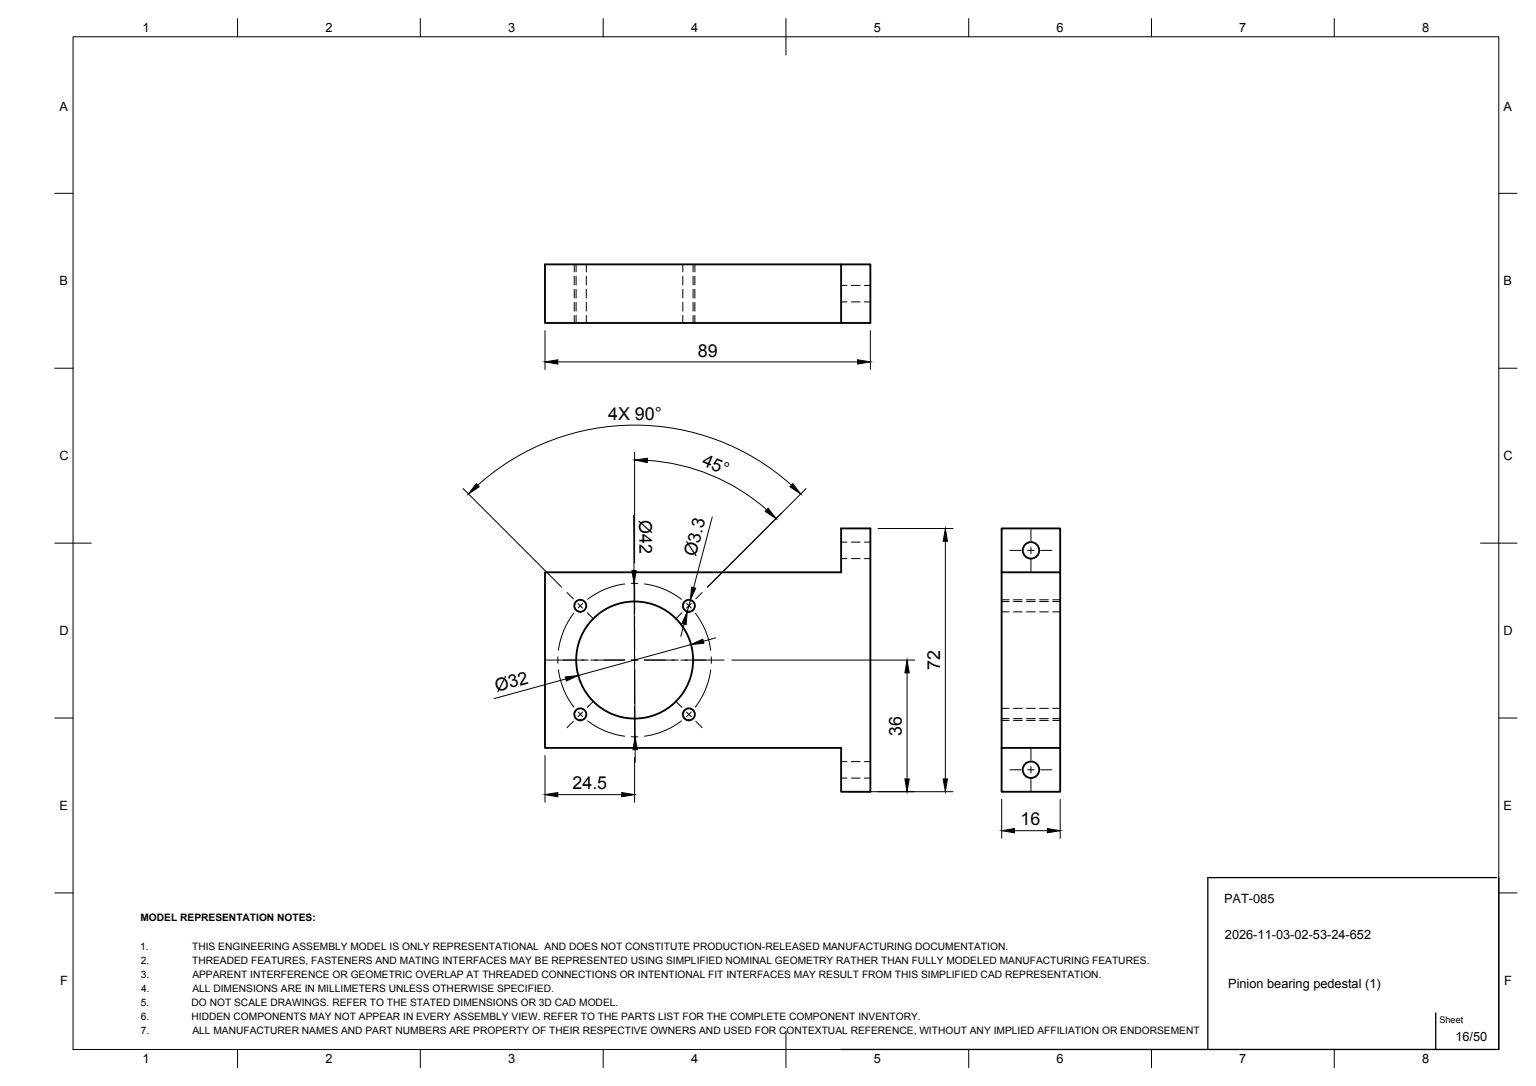
ISO-10303-21;
HEADER;
/* Generated by software containing ST-Developer
 * from STEP Tools, Inc. (www.steptools.com) 
 */

FILE_DESCRIPTION(
/* description */ ('Rack and pinion manual slide'),
/* implementation_level */ '2;1');

FILE_NAME(
/* name */ 'Pinion bearing pedestal (1).step',
/* time_stamp */ '2026-10-28T03:22:49-07:00',
/* author */ (''),
/* organization */ (''),
/* preprocessor_version */ 'ST-DEVELOPER v20.2',
/* originating_system */ 'Autodesk Translation Framework v15.17.0.0',
/* authorisation */ '');

FILE_SCHEMA (('AUTOMOTIVE_DESIGN { 1 0 10303 214 3 1 1 }'));
ENDSEC;

DATA;
#10=MECHANICAL_DESIGN_GEOMETRIC_PRESENTATION_REPRESENTATION('',(#743),#34851);
#651=SHAPE_REPRESENTATION_RELATIONSHIP('SRR','None',#35086,#697);
#697=ADVANCED_BREP_SHAPE_REPRESENTATION('',(#796),#34811);
#743=STYLED_ITEM('',(#35411),#796);
#796=MANIFOLD_SOLID_BREP('Body1',#13763);
#921=FACE_BOUND('',#2487,.T.);
#922=FACE_BOUND('',#2489,.T.);
#923=FACE_BOUND('',#2493,.T.);
#924=FACE_BOUND('',#2494,.T.);
#925=FACE_BOUND('',#2495,.T.);
#926=FACE_BOUND('',#2496,.T.);
#927=FACE_BOUND('',#2497,.T.);
#928=FACE_BOUND('',#2500,.T.);
#929=FACE_BOUND('',#2501,.T.);
#930=FACE_BOUND('',#2502,.T.);
#931=FACE_BOUND('',#2503,.T.);
#932=FACE_BOUND('',#2504,.T.);
#933=FACE_BOUND('',#2508,.T.);
#934=FACE_BOUND('',#2509,.T.);
#1112=PLANE('',#14567);
#1113=PLANE('',#14568);
#1114=PLANE('',#14569);
#1115=PLANE('',#14570);
#1116=PLANE('',#14571);
#1117=PLANE('',#14572);
#1118=PLANE('',#14573);
#1119=PLANE('',#14574);
#1120=PLANE('',#14575);
#1121=PLANE('',#14576);
#1652=FACE_OUTER_BOUND('',#2479,.T.);
#1653=FACE_OUTER_BOUND('',#2480,.T.);
#1654=FACE_OUTER_BOUND('',#2481,.T.);
#1655=FACE_OUTER_BOUND('',#2482,.T.);
#1656=FACE_OUTER_BOUND('',#2483,.T.);
#1657=FACE_OUTER_BOUND('',#2484,.T.);
#1658=FACE_OUTER_BOUND('',#2485,.T.);
#1659=FACE_OUTER_BOUND('',#2486,.T.);
#1660=FACE_OUTER_BOUND('',#2488,.T.);
#1661=FACE_OUTER_BOUND('',#2490,.T.);
#1662=FACE_OUTER_BOUND('',#2491,.T.);
#1663=FACE_OUTER_BOUND('',#2492,.T.);
#1664=FACE_OUTER_BOUND('',#2498,.T.);
#1665=FACE_OUTER_BOUND('',#2499,.T.);
#1666=FACE_OUTER_BOUND('',#2505,.T.);
#1667=FACE_OUTER_BOUND('',#2506,.T.);
#1668=FACE_OUTER_BOUND('',#2507,.T.);
#2479=EDGE_LOOP('',(#9768,#9769,#9770,#9771));
#2480=EDGE_LOOP('',(#9772,#9773,#9774,#9775));
#2481=EDGE_LOOP('',(#9776,#9777,#9778,#9779));
#2482=EDGE_LOOP('',(#9780,#9781,#9782,#9783));
#2483=EDGE_LOOP('',(#9784,#9785,#9786,#9787));
#2484=EDGE_LOOP('',(#9788,#9789,#9790,#9791));
#2485=EDGE_LOOP('',(#9792,#9793,#9794,#9795));
#2486=EDGE_LOOP('',(#9796,#9797,#9798,#9799));
#2487=EDGE_LOOP('',(#9800));
#2488=EDGE_LOOP('',(#9801,#9802,#9803,#9804));
#2489=EDGE_LOOP('',(#9805));
#2490=EDGE_LOOP('',(#9806,#9807,#9808,#9809));
#2491=EDGE_LOOP('',(#9810,#9811,#9812,#9813));
#2492=EDGE_LOOP('',(#9814,#9815,#9816,#9817,#9818,#9819,#9820,#9821));
#2493=EDGE_LOOP('',(#9822));
#2494=EDGE_LOOP('',(#9823));
#2495=EDGE_LOOP('',(#9824));
#2496=EDGE_LOOP('',(#9825));
#2497=EDGE_LOOP('',(#9826));
#2498=EDGE_LOOP('',(#9827,#9828,#9829,#9830));
#2499=EDGE_LOOP('',(#9831,#9832,#9833,#9834,#9835,#9836,#9837,#9838));
#2500=EDGE_LOOP('',(#9839));
#2501=EDGE_LOOP('',(#9840));
#2502=EDGE_LOOP('',(#9841));
#2503=EDGE_LOOP('',(#9842));
#2504=EDGE_LOOP('',(#9843));
#2505=EDGE_LOOP('',(#9844,#9845,#9846,#9847));
#2506=EDGE_LOOP('',(#9848,#9849,#9850,#9851));
#2507=EDGE_LOOP('',(#9852,#9853,#9854,#9855));
#2508=EDGE_LOOP('',(#9856));
#2509=EDGE_LOOP('',(#9857));
#3393=LINE('',#20037,#4684);
#3394=LINE('',#20043,#4685);
#3395=LINE('',#20049,#4686);
#3396=LINE('',#20055,#4687);
#3397=LINE('',#20061,#4688);
#3398=LINE('',#20067,#4689);
#3399=LINE('',#20073,#4690);
#3400=LINE('',#20078,#4691);
#3401=LINE('',#20080,#4692);
#3402=LINE('',#20082,#4693);
#3403=LINE('',#20083,#4694);
#3404=LINE('',#20087,#4695);
#3405=LINE('',#20089,#4696);
#3406=LINE('',#20091,#4697);
#3407=LINE('',#20092,#4698);
#3408=LINE('',#20095,#4699);
#3409=LINE('',#20097,#4700);
#3410=LINE('',#20098,#4701);
#3411=LINE('',#20101,#4702);
#3412=LINE('',#20103,#4703);
#3413=LINE('',#20104,#4704);
#3414=LINE('',#20107,#4705);
#3415=LINE('',#20109,#4706);
#3416=LINE('',#20110,#4707);
#3417=LINE('',#20111,#4708);
#3418=LINE('',#20114,#4709);
#3419=LINE('',#20115,#4710);
#3420=LINE('',#20118,#4711);
#3421=LINE('',#20119,#4712);
#3422=LINE('',#20120,#4713);
#3423=LINE('',#20122,#4714);
#4684=VECTOR('',#16231,0.225);
#4685=VECTOR('',#16238,0.225);
#4686=VECTOR('',#16245,0.164999999999999);
#4687=VECTOR('',#16252,0.164999999999999);
#4688=VECTOR('',#16259,0.164999999999999);
#4689=VECTOR('',#16266,0.164999999999999);
#4690=VECTOR('',#16273,1.6);
#4691=VECTOR('',#16278,1.);
#4692=VECTOR('',#16279,1.);
#4693=VECTOR('',#16280,1.);
#4694=VECTOR('',#16281,1.);
#4695=VECTOR('',#16284,1.);
#4696=VECTOR('',#16285,1.);
#4697=VECTOR('',#16286,1.);
#4698=VECTOR('',#16287,1.);
#4699=VECTOR('',#16290,1.);
#4700=VECTOR('',#16291,1.);
#4701=VECTOR('',#16292,1.);
#4702=VECTOR('',#16295,1.);
#4703=VECTOR('',#16296,1.);
#4704=VECTOR('',#16297,1.);
#4705=VECTOR('',#16300,1.);
#4706=VECTOR('',#16301,1.);
#4707=VECTOR('',#16302,1.);
#4708=VECTOR('',#16303,1.);
#4709=VECTOR('',#16306,1.);
#4710=VECTOR('',#16307,1.);
#4711=VECTOR('',#16310,1.);
#4712=VECTOR('',#16311,1.);
#4713=VECTOR('',#16312,1.);
#4714=VECTOR('',#16315,1.);
#5904=CIRCLE('',#14547,0.225);
#5905=CIRCLE('',#14548,0.225);
#5906=CIRCLE('',#14550,0.225);
#5907=CIRCLE('',#14551,0.225);
#5908=CIRCLE('',#14553,0.164999999999999);
#5909=CIRCLE('',#14554,0.164999999999999);
#5910=CIRCLE('',#14556,0.164999999999999);
#5911=CIRCLE('',#14557,0.164999999999999);
#5912=CIRCLE('',#14559,0.164999999999999);
#5913=CIRCLE('',#14560,0.164999999999999);
#5914=CIRCLE('',#14562,0.164999999999999);
#5915=CIRCLE('',#14563,0.164999999999999);
#5916=CIRCLE('',#14565,1.6);
#5917=CIRCLE('',#14566,1.6);
#6402=VERTEX_POINT('',#20034);
#6403=VERTEX_POINT('',#20036);
#6404=VERTEX_POINT('',#20040);
#6405=VERTEX_POINT('',#20042);
#6406=VERTEX_POINT('',#20046);
#6407=VERTEX_POINT('',#20048);
#6408=VERTEX_POINT('',#20052);
#6409=VERTEX_POINT('',#20054);
#6410=VERTEX_POINT('',#20058);
#6411=VERTEX_POINT('',#20060);
#6412=VERTEX_POINT('',#20064);
#6413=VERTEX_POINT('',#20066);
#6414=VERTEX_POINT('',#20070);
#6415=VERTEX_POINT('',#20072);
#6416=VERTEX_POINT('',#20076);
#6417=VERTEX_POINT('',#20077);
#6418=VERTEX_POINT('',#20079);
#6419=VERTEX_POINT('',#20081);
#6420=VERTEX_POINT('',#20085);
#6421=VERTEX_POINT('',#20086);
#6422=VERTEX_POINT('',#20088);
#6423=VERTEX_POINT('',#20090);
#6424=VERTEX_POINT('',#20094);
#6425=VERTEX_POINT('',#20096);
#6426=VERTEX_POINT('',#20100);
#6427=VERTEX_POINT('',#20102);
#6428=VERTEX_POINT('',#20106);
#6429=VERTEX_POINT('',#20108);
#6430=VERTEX_POINT('',#20113);
#6431=VERTEX_POINT('',#20117);
#7696=EDGE_CURVE('',#6402,#6402,#5904,.T.);
#7697=EDGE_CURVE('',#6402,#6403,#3393,.T.);
#7698=EDGE_CURVE('',#6403,#6403,#5905,.T.);
#7699=EDGE_CURVE('',#6404,#6404,#5906,.T.);
#7700=EDGE_CURVE('',#6404,#6405,#3394,.T.);
#7701=EDGE_CURVE('',#6405,#6405,#5907,.T.);
#7702=EDGE_CURVE('',#6406,#6406,#5908,.T.);
#7703=EDGE_CURVE('',#6406,#6407,#3395,.T.);
#7704=EDGE_CURVE('',#6407,#6407,#5909,.T.);
#7705=EDGE_CURVE('',#6408,#6408,#5910,.T.);
#7706=EDGE_CURVE('',#6408,#6409,#3396,.T.);
#7707=EDGE_CURVE('',#6409,#6409,#5911,.T.);
#7708=EDGE_CURVE('',#6410,#6410,#5912,.T.);
#7709=EDGE_CURVE('',#6410,#6411,#3397,.T.);
#7710=EDGE_CURVE('',#6411,#6411,#5913,.T.);
#7711=EDGE_CURVE('',#6412,#6412,#5914,.T.);
#7712=EDGE_CURVE('',#6412,#6413,#3398,.T.);
#7713=EDGE_CURVE('',#6413,#6413,#5915,.T.);
#7714=EDGE_CURVE('',#6414,#6414,#5916,.T.);
#7715=EDGE_CURVE('',#6414,#6415,#3399,.T.);
#7716=EDGE_CURVE('',#6415,#6415,#5917,.T.);
#7717=EDGE_CURVE('',#6416,#6417,#3400,.T.);
#7718=EDGE_CURVE('',#6418,#6416,#3401,.T.);
#7719=EDGE_CURVE('',#6418,#6419,#3402,.T.);
#7720=EDGE_CURVE('',#6417,#6419,#3403,.T.);
#7721=EDGE_CURVE('',#6420,#6421,#3404,.T.);
#7722=EDGE_CURVE('',#6422,#6420,#3405,.T.);
#7723=EDGE_CURVE('',#6423,#6422,#3406,.T.);
#7724=EDGE_CURVE('',#6421,#6423,#3407,.T.);
#7725=EDGE_CURVE('',#6423,#6424,#3408,.T.);
#7726=EDGE_CURVE('',#6425,#6422,#3409,.T.);
#7727=EDGE_CURVE('',#6424,#6425,#3410,.T.);
#7728=EDGE_CURVE('',#6426,#6418,#3411,.T.);
#7729=EDGE_CURVE('',#6426,#6427,#3412,.T.);
#7730=EDGE_CURVE('',#6419,#6427,#3413,.T.);
#7731=EDGE_CURVE('',#6416,#6428,#3414,.T.);
#7732=EDGE_CURVE('',#6429,#6428,#3415,.T.);
#7733=EDGE_CURVE('',#6421,#6429,#3416,.T.);
#7734=EDGE_CURVE('',#6424,#6426,#3417,.T.);
#7735=EDGE_CURVE('',#6417,#6430,#3418,.T.);
#7736=EDGE_CURVE('',#6428,#6430,#3419,.T.);
#7737=EDGE_CURVE('',#6420,#6431,#3420,.T.);
#7738=EDGE_CURVE('',#6430,#6431,#3421,.T.);
#7739=EDGE_CURVE('',#6427,#6425,#3422,.T.);
#7740=EDGE_CURVE('',#6431,#6429,#3423,.T.);
#9768=ORIENTED_EDGE('',*,*,#7696,.F.);
#9769=ORIENTED_EDGE('',*,*,#7697,.T.);
#9770=ORIENTED_EDGE('',*,*,#7698,.F.);
#9771=ORIENTED_EDGE('',*,*,#7697,.F.);
#9772=ORIENTED_EDGE('',*,*,#7699,.F.);
#9773=ORIENTED_EDGE('',*,*,#7700,.T.);
#9774=ORIENTED_EDGE('',*,*,#7701,.F.);
#9775=ORIENTED_EDGE('',*,*,#7700,.F.);
#9776=ORIENTED_EDGE('',*,*,#7702,.F.);
#9777=ORIENTED_EDGE('',*,*,#7703,.T.);
#9778=ORIENTED_EDGE('',*,*,#7704,.F.);
#9779=ORIENTED_EDGE('',*,*,#7703,.F.);
#9780=ORIENTED_EDGE('',*,*,#7705,.F.);
#9781=ORIENTED_EDGE('',*,*,#7706,.T.);
#9782=ORIENTED_EDGE('',*,*,#7707,.F.);
#9783=ORIENTED_EDGE('',*,*,#7706,.F.);
#9784=ORIENTED_EDGE('',*,*,#7708,.F.);
#9785=ORIENTED_EDGE('',*,*,#7709,.T.);
#9786=ORIENTED_EDGE('',*,*,#7710,.F.);
#9787=ORIENTED_EDGE('',*,*,#7709,.F.);
#9788=ORIENTED_EDGE('',*,*,#7711,.F.);
#9789=ORIENTED_EDGE('',*,*,#7712,.T.);
#9790=ORIENTED_EDGE('',*,*,#7713,.F.);
#9791=ORIENTED_EDGE('',*,*,#7712,.F.);
#9792=ORIENTED_EDGE('',*,*,#7714,.F.);
#9793=ORIENTED_EDGE('',*,*,#7715,.T.);
#9794=ORIENTED_EDGE('',*,*,#7716,.F.);
#9795=ORIENTED_EDGE('',*,*,#7715,.F.);
#9796=ORIENTED_EDGE('',*,*,#7717,.F.);
#9797=ORIENTED_EDGE('',*,*,#7718,.F.);
#9798=ORIENTED_EDGE('',*,*,#7719,.T.);
#9799=ORIENTED_EDGE('',*,*,#7720,.F.);
#9800=ORIENTED_EDGE('',*,*,#7701,.T.);
#9801=ORIENTED_EDGE('',*,*,#7721,.F.);
#9802=ORIENTED_EDGE('',*,*,#7722,.F.);
#9803=ORIENTED_EDGE('',*,*,#7723,.F.);
#9804=ORIENTED_EDGE('',*,*,#7724,.F.);
#9805=ORIENTED_EDGE('',*,*,#7698,.T.);
#9806=ORIENTED_EDGE('',*,*,#7725,.F.);
#9807=ORIENTED_EDGE('',*,*,#7723,.T.);
#9808=ORIENTED_EDGE('',*,*,#7726,.F.);
#9809=ORIENTED_EDGE('',*,*,#7727,.F.);
#9810=ORIENTED_EDGE('',*,*,#7728,.F.);
#9811=ORIENTED_EDGE('',*,*,#7729,.T.);
#9812=ORIENTED_EDGE('',*,*,#7730,.F.);
#9813=ORIENTED_EDGE('',*,*,#7719,.F.);
#9814=ORIENTED_EDGE('',*,*,#7731,.T.);
#9815=ORIENTED_EDGE('',*,*,#7732,.F.);
#9816=ORIENTED_EDGE('',*,*,#7733,.F.);
#9817=ORIENTED_EDGE('',*,*,#7724,.T.);
#9818=ORIENTED_EDGE('',*,*,#7725,.T.);
#9819=ORIENTED_EDGE('',*,*,#7734,.T.);
#9820=ORIENTED_EDGE('',*,*,#7728,.T.);
#9821=ORIENTED_EDGE('',*,*,#7718,.T.);
#9822=ORIENTED_EDGE('',*,*,#7714,.T.);
#9823=ORIENTED_EDGE('',*,*,#7711,.T.);
#9824=ORIENTED_EDGE('',*,*,#7708,.T.);
#9825=ORIENTED_EDGE('',*,*,#7705,.T.);
#9826=ORIENTED_EDGE('',*,*,#7702,.T.);
#9827=ORIENTED_EDGE('',*,*,#7717,.T.);
#9828=ORIENTED_EDGE('',*,*,#7735,.T.);
#9829=ORIENTED_EDGE('',*,*,#7736,.F.);
#9830=ORIENTED_EDGE('',*,*,#7731,.F.);
#9831=ORIENTED_EDGE('',*,*,#7737,.T.);
#9832=ORIENTED_EDGE('',*,*,#7738,.F.);
#9833=ORIENTED_EDGE('',*,*,#7735,.F.);
#9834=ORIENTED_EDGE('',*,*,#7720,.T.);
#9835=ORIENTED_EDGE('',*,*,#7730,.T.);
#9836=ORIENTED_EDGE('',*,*,#7739,.T.);
#9837=ORIENTED_EDGE('',*,*,#7726,.T.);
#9838=ORIENTED_EDGE('',*,*,#7722,.T.);
#9839=ORIENTED_EDGE('',*,*,#7716,.T.);
#9840=ORIENTED_EDGE('',*,*,#7713,.T.);
#9841=ORIENTED_EDGE('',*,*,#7710,.T.);
#9842=ORIENTED_EDGE('',*,*,#7707,.T.);
#9843=ORIENTED_EDGE('',*,*,#7704,.T.);
#9844=ORIENTED_EDGE('',*,*,#7721,.T.);
#9845=ORIENTED_EDGE('',*,*,#7733,.T.);
#9846=ORIENTED_EDGE('',*,*,#7740,.F.);
#9847=ORIENTED_EDGE('',*,*,#7737,.F.);
#9848=ORIENTED_EDGE('',*,*,#7740,.T.);
#9849=ORIENTED_EDGE('',*,*,#7732,.T.);
#9850=ORIENTED_EDGE('',*,*,#7736,.T.);
#9851=ORIENTED_EDGE('',*,*,#7738,.T.);
#9852=ORIENTED_EDGE('',*,*,#7739,.F.);
#9853=ORIENTED_EDGE('',*,*,#7729,.F.);
#9854=ORIENTED_EDGE('',*,*,#7734,.F.);
#9855=ORIENTED_EDGE('',*,*,#7727,.T.);
#9856=ORIENTED_EDGE('',*,*,#7696,.T.);
#9857=ORIENTED_EDGE('',*,*,#7699,.T.);
#12893=CYLINDRICAL_SURFACE('',#14546,0.225);
#12894=CYLINDRICAL_SURFACE('',#14549,0.225);
#12895=CYLINDRICAL_SURFACE('',#14552,0.164999999999999);
#12896=CYLINDRICAL_SURFACE('',#14555,0.164999999999999);
#12897=CYLINDRICAL_SURFACE('',#14558,0.164999999999999);
#12898=CYLINDRICAL_SURFACE('',#14561,0.164999999999999);
#12899=CYLINDRICAL_SURFACE('',#14564,1.6);
#13130=ADVANCED_FACE('',(#1652),#12893,.F.);
#13131=ADVANCED_FACE('',(#1653),#12894,.F.);
#13132=ADVANCED_FACE('',(#1654),#12895,.F.);
#13133=ADVANCED_FACE('',(#1655),#12896,.F.);
#13134=ADVANCED_FACE('',(#1656),#12897,.F.);
#13135=ADVANCED_FACE('',(#1657),#12898,.F.);
#13136=ADVANCED_FACE('',(#1658),#12899,.F.);
#13137=ADVANCED_FACE('',(#1659,#921),#1112,.T.);
#13138=ADVANCED_FACE('',(#1660,#922),#1113,.T.);
#13139=ADVANCED_FACE('',(#1661),#1114,.T.);
#13140=ADVANCED_FACE('',(#1662),#1115,.T.);
#13141=ADVANCED_FACE('',(#1663,#923,#924,#925,#926,#927),#1116,.T.);
#13142=ADVANCED_FACE('',(#1664),#1117,.T.);
#13143=ADVANCED_FACE('',(#1665,#928,#929,#930,#931,#932),#1118,.T.);
#13144=ADVANCED_FACE('',(#1666),#1119,.T.);
#13145=ADVANCED_FACE('',(#1667),#1120,.T.);
#13146=ADVANCED_FACE('',(#1668,#933,#934),#1121,.F.);
#13763=CLOSED_SHELL('',(#13130,#13131,#13132,#13133,#13134,#13135,#13136,
#13137,#13138,#13139,#13140,#13141,#13142,#13143,#13144,#13145,#13146));
#14545=AXIS2_PLACEMENT_3D('',#20032,#16225,#16226);
#14546=AXIS2_PLACEMENT_3D('',#20033,#16227,#16228);
#14547=AXIS2_PLACEMENT_3D('',#20035,#16229,#16230);
#14548=AXIS2_PLACEMENT_3D('',#20038,#16232,#16233);
#14549=AXIS2_PLACEMENT_3D('',#20039,#16234,#16235);
#14550=AXIS2_PLACEMENT_3D('',#20041,#16236,#16237);
#14551=AXIS2_PLACEMENT_3D('',#20044,#16239,#16240);
#14552=AXIS2_PLACEMENT_3D('',#20045,#16241,#16242);
#14553=AXIS2_PLACEMENT_3D('',#20047,#16243,#16244);
#14554=AXIS2_PLACEMENT_3D('',#20050,#16246,#16247);
#14555=AXIS2_PLACEMENT_3D('',#20051,#16248,#16249);
#14556=AXIS2_PLACEMENT_3D('',#20053,#16250,#16251);
#14557=AXIS2_PLACEMENT_3D('',#20056,#16253,#16254);
#14558=AXIS2_PLACEMENT_3D('',#20057,#16255,#16256);
#14559=AXIS2_PLACEMENT_3D('',#20059,#16257,#16258);
#14560=AXIS2_PLACEMENT_3D('',#20062,#16260,#16261);
#14561=AXIS2_PLACEMENT_3D('',#20063,#16262,#16263);
#14562=AXIS2_PLACEMENT_3D('',#20065,#16264,#16265);
#14563=AXIS2_PLACEMENT_3D('',#20068,#16267,#16268);
#14564=AXIS2_PLACEMENT_3D('',#20069,#16269,#16270);
#14565=AXIS2_PLACEMENT_3D('',#20071,#16271,#16272);
#14566=AXIS2_PLACEMENT_3D('',#20074,#16274,#16275);
#14567=AXIS2_PLACEMENT_3D('',#20075,#16276,#16277);
#14568=AXIS2_PLACEMENT_3D('',#20084,#16282,#16283);
#14569=AXIS2_PLACEMENT_3D('',#20093,#16288,#16289);
#14570=AXIS2_PLACEMENT_3D('',#20099,#16293,#16294);
#14571=AXIS2_PLACEMENT_3D('',#20105,#16298,#16299);
#14572=AXIS2_PLACEMENT_3D('',#20112,#16304,#16305);
#14573=AXIS2_PLACEMENT_3D('',#20116,#16308,#16309);
#14574=AXIS2_PLACEMENT_3D('',#20121,#16313,#16314);
#14575=AXIS2_PLACEMENT_3D('',#20123,#16316,#16317);
#14576=AXIS2_PLACEMENT_3D('',#20124,#16318,#16319);
#16225=DIRECTION('axis',(0.,0.,1.));
#16226=DIRECTION('refdir',(1.,0.,0.));
#16227=DIRECTION('center_axis',(0.,0.,1.));
#16228=DIRECTION('ref_axis',(1.,0.,0.));
#16229=DIRECTION('center_axis',(0.,0.,1.));
#16230=DIRECTION('ref_axis',(1.,0.,0.));
#16231=DIRECTION('',(0.,0.,1.));
#16232=DIRECTION('center_axis',(0.,0.,-1.));
#16233=DIRECTION('ref_axis',(1.,0.,0.));
#16234=DIRECTION('center_axis',(0.,0.,1.));
#16235=DIRECTION('ref_axis',(1.,0.,0.));
#16236=DIRECTION('center_axis',(0.,0.,1.));
#16237=DIRECTION('ref_axis',(1.,0.,0.));
#16238=DIRECTION('',(0.,0.,1.));
#16239=DIRECTION('center_axis',(0.,0.,-1.));
#16240=DIRECTION('ref_axis',(1.,0.,0.));
#16241=DIRECTION('center_axis',(0.,1.,0.));
#16242=DIRECTION('ref_axis',(1.,0.,0.));
#16243=DIRECTION('center_axis',(0.,1.,0.));
#16244=DIRECTION('ref_axis',(1.,0.,0.));
#16245=DIRECTION('',(0.,1.,0.));
#16246=DIRECTION('center_axis',(0.,-1.,0.));
#16247=DIRECTION('ref_axis',(1.,0.,0.));
#16248=DIRECTION('center_axis',(0.,1.,0.));
#16249=DIRECTION('ref_axis',(1.,0.,0.));
#16250=DIRECTION('center_axis',(0.,1.,0.));
#16251=DIRECTION('ref_axis',(1.,0.,0.));
#16252=DIRECTION('',(0.,1.,0.));
#16253=DIRECTION('center_axis',(0.,-1.,0.));
#16254=DIRECTION('ref_axis',(1.,0.,0.));
#16255=DIRECTION('center_axis',(0.,1.,0.));
#16256=DIRECTION('ref_axis',(1.,0.,0.));
#16257=DIRECTION('center_axis',(0.,1.,0.));
#16258=DIRECTION('ref_axis',(1.,0.,0.));
#16259=DIRECTION('',(0.,1.,0.));
#16260=DIRECTION('center_axis',(0.,-1.,0.));
#16261=DIRECTION('ref_axis',(1.,0.,0.));
#16262=DIRECTION('center_axis',(0.,1.,0.));
#16263=DIRECTION('ref_axis',(1.,0.,0.));
#16264=DIRECTION('center_axis',(0.,1.,0.));
#16265=DIRECTION('ref_axis',(1.,0.,0.));
#16266=DIRECTION('',(0.,1.,0.));
#16267=DIRECTION('center_axis',(0.,-1.,0.));
#16268=DIRECTION('ref_axis',(1.,0.,0.));
#16269=DIRECTION('center_axis',(0.,1.,0.));
#16270=DIRECTION('ref_axis',(1.,0.,0.));
#16271=DIRECTION('center_axis',(0.,1.,0.));
#16272=DIRECTION('ref_axis',(1.,0.,0.));
#16273=DIRECTION('',(0.,1.,0.));
#16274=DIRECTION('center_axis',(0.,-1.,0.));
#16275=DIRECTION('ref_axis',(1.,0.,0.));
#16276=DIRECTION('center_axis',(0.,0.,1.));
#16277=DIRECTION('ref_axis',(1.,0.,0.));
#16278=DIRECTION('',(0.,1.,0.));
#16279=DIRECTION('',(-1.,0.,0.));
#16280=DIRECTION('',(0.,1.,0.));
#16281=DIRECTION('',(1.,0.,0.));
#16282=DIRECTION('center_axis',(0.,0.,1.));
#16283=DIRECTION('ref_axis',(1.,0.,0.));
#16284=DIRECTION('',(0.,-1.,0.));
#16285=DIRECTION('',(1.,0.,0.));
#16286=DIRECTION('',(0.,1.,0.));
#16287=DIRECTION('',(-1.,0.,0.));
#16288=DIRECTION('center_axis',(-1.,0.,0.));
#16289=DIRECTION('ref_axis',(0.,0.,1.));
#16290=DIRECTION('',(0.,0.,-1.));
#16291=DIRECTION('',(0.,0.,1.));
#16292=DIRECTION('',(0.,1.,0.));
#16293=DIRECTION('center_axis',(1.,0.,0.));
#16294=DIRECTION('ref_axis',(0.,0.,-1.));
#16295=DIRECTION('',(0.,0.,1.));
#16296=DIRECTION('',(0.,1.,0.));
#16297=DIRECTION('',(0.,0.,-1.));
#16298=DIRECTION('center_axis',(0.,-1.,0.));
#16299=DIRECTION('ref_axis',(1.,0.,0.));
#16300=DIRECTION('',(0.,0.,1.));
#16301=DIRECTION('',(1.,0.,0.));
#16302=DIRECTION('',(0.,0.,1.));
#16303=DIRECTION('',(1.,0.,0.));
#16304=DIRECTION('center_axis',(1.,0.,0.));
#16305=DIRECTION('ref_axis',(0.,1.,0.));
#16306=DIRECTION('',(0.,0.,1.));
#16307=DIRECTION('',(0.,1.,0.));
#16308=DIRECTION('center_axis',(0.,1.,0.));
#16309=DIRECTION('ref_axis',(-1.,0.,0.));
#16310=DIRECTION('',(0.,0.,1.));
#16311=DIRECTION('',(-1.,0.,0.));
#16312=DIRECTION('',(-1.,0.,0.));
#16313=DIRECTION('center_axis',(-1.,0.,0.));
#16314=DIRECTION('ref_axis',(0.,-1.,0.));
#16315=DIRECTION('',(0.,-1.,0.));
#16316=DIRECTION('center_axis',(0.,0.,1.));
#16317=DIRECTION('ref_axis',(1.,0.,0.));
#16318=DIRECTION('center_axis',(0.,0.,1.));
#16319=DIRECTION('ref_axis',(1.,0.,0.));
#20032=CARTESIAN_POINT('',(0.,0.,0.));
#20033=CARTESIAN_POINT('Origin',(8.,4.2,3.7));
#20034=CARTESIAN_POINT('',(7.775,4.2,3.8));
#20035=CARTESIAN_POINT('Origin',(8.,4.2,3.8));
#20036=CARTESIAN_POINT('',(7.775,4.2,4.6));
#20037=CARTESIAN_POINT('',(7.775,4.2,3.7));
#20038=CARTESIAN_POINT('Origin',(8.,4.2,4.6));
#20039=CARTESIAN_POINT('Origin',(14.,4.2,3.7));
#20040=CARTESIAN_POINT('',(13.775,4.2,3.8));
#20041=CARTESIAN_POINT('Origin',(14.,4.2,3.8));
#20042=CARTESIAN_POINT('',(13.775,4.2,4.6));
#20043=CARTESIAN_POINT('',(13.775,4.2,3.7));
#20044=CARTESIAN_POINT('Origin',(14.,4.2,4.6));
#20045=CARTESIAN_POINT('Origin',(9.51507575950825,3.3,8.76507575950825));
#20046=CARTESIAN_POINT('',(9.35007575950825,3.4,8.76507575950825));
#20047=CARTESIAN_POINT('Origin',(9.51507575950825,3.4,8.76507575950825));
#20048=CARTESIAN_POINT('',(9.35007575950825,5.,8.76507575950825));
#20049=CARTESIAN_POINT('',(9.35007575950825,3.3,8.76507575950825));
#20050=CARTESIAN_POINT('Origin',(9.51507575950825,5.,8.76507575950825));
#20051=CARTESIAN_POINT('Origin',(9.51507575950825,3.3,11.7349242404918));
#20052=CARTESIAN_POINT('',(9.35007575950825,3.4,11.7349242404918));
#20053=CARTESIAN_POINT('Origin',(9.51507575950825,3.4,11.7349242404918));
#20054=CARTESIAN_POINT('',(9.35007575950825,5.,11.7349242404918));
#20055=CARTESIAN_POINT('',(9.35007575950825,3.3,11.7349242404918));
#20056=CARTESIAN_POINT('Origin',(9.51507575950825,5.,11.7349242404918));
#20057=CARTESIAN_POINT('Origin',(12.4849242404918,3.3,11.7349242404918));
#20058=CARTESIAN_POINT('',(12.3199242404918,3.4,11.7349242404918));
#20059=CARTESIAN_POINT('Origin',(12.4849242404918,3.4,11.7349242404918));
#20060=CARTESIAN_POINT('',(12.3199242404918,5.,11.7349242404918));
#20061=CARTESIAN_POINT('',(12.3199242404918,3.3,11.7349242404918));
#20062=CARTESIAN_POINT('Origin',(12.4849242404918,5.,11.7349242404918));
#20063=CARTESIAN_POINT('Origin',(12.4849242404917,3.3,8.76507575950825));
#20064=CARTESIAN_POINT('',(12.3199242404917,3.4,8.76507575950825));
#20065=CARTESIAN_POINT('Origin',(12.4849242404917,3.4,8.76507575950825));
#20066=CARTESIAN_POINT('',(12.3199242404917,5.,8.76507575950825));
#20067=CARTESIAN_POINT('',(12.3199242404917,3.3,8.76507575950825));
#20068=CARTESIAN_POINT('Origin',(12.4849242404917,5.,8.76507575950825));
#20069=CARTESIAN_POINT('Origin',(11.,3.3,10.25));
#20070=CARTESIAN_POINT('',(9.4,3.4,10.25));
#20071=CARTESIAN_POINT('Origin',(11.,3.4,10.25));
#20072=CARTESIAN_POINT('',(9.4,5.,10.25));
#20073=CARTESIAN_POINT('',(9.4,3.3,10.25));
#20074=CARTESIAN_POINT('Origin',(11.,5.,10.25));
#20075=CARTESIAN_POINT('Origin',(7.4,3.4,4.6));
#20076=CARTESIAN_POINT('',(13.4,3.4,4.6));
#20077=CARTESIAN_POINT('',(13.4,5.,4.6));
#20078=CARTESIAN_POINT('',(13.4,3.4,4.6));
#20079=CARTESIAN_POINT('',(14.6,3.4,4.6));
#20080=CARTESIAN_POINT('',(14.6,3.4,4.6));
#20081=CARTESIAN_POINT('',(14.6,5.,4.6));
#20082=CARTESIAN_POINT('',(14.6,3.4,4.6));
#20083=CARTESIAN_POINT('',(14.6,5.,4.6));
#20084=CARTESIAN_POINT('Origin',(7.4,3.4,4.6));
#20085=CARTESIAN_POINT('',(8.6,5.,4.6));
#20086=CARTESIAN_POINT('',(8.6,3.4,4.6));
#20087=CARTESIAN_POINT('',(8.6,4.2,4.6));
#20088=CARTESIAN_POINT('',(7.4,5.,4.6));
#20089=CARTESIAN_POINT('',(14.6,5.,4.6));
#20090=CARTESIAN_POINT('',(7.4,3.4,4.6));
#20091=CARTESIAN_POINT('',(7.4,3.4,4.6));
#20092=CARTESIAN_POINT('',(14.6,3.4,4.6));
#20093=CARTESIAN_POINT('Origin',(7.4,3.4,3.8));
#20094=CARTESIAN_POINT('',(7.4,3.4,3.8));
#20095=CARTESIAN_POINT('',(7.4,3.4,4.6));
#20096=CARTESIAN_POINT('',(7.4,5.,3.8));
#20097=CARTESIAN_POINT('',(7.4,5.,4.6));
#20098=CARTESIAN_POINT('',(7.4,3.4,3.8));
#20099=CARTESIAN_POINT('Origin',(14.6,3.4,4.6));
#20100=CARTESIAN_POINT('',(14.6,3.4,3.8));
#20101=CARTESIAN_POINT('',(14.6,3.4,3.8));
#20102=CARTESIAN_POINT('',(14.6,5.,3.8));
#20103=CARTESIAN_POINT('',(14.6,3.4,3.8));
#20104=CARTESIAN_POINT('',(14.6,5.,3.8));
#20105=CARTESIAN_POINT('Origin',(8.6,3.4,3.8));
#20106=CARTESIAN_POINT('',(13.4,3.4,12.7));
#20107=CARTESIAN_POINT('',(13.4,3.4,3.8));
#20108=CARTESIAN_POINT('',(8.6,3.4,12.7));
#20109=CARTESIAN_POINT('',(8.6,3.4,12.7));
#20110=CARTESIAN_POINT('',(8.6,3.4,3.8));
#20111=CARTESIAN_POINT('',(7.4,3.4,3.8));
#20112=CARTESIAN_POINT('Origin',(13.4,3.4,3.8));
#20113=CARTESIAN_POINT('',(13.4,5.,12.7));
#20114=CARTESIAN_POINT('',(13.4,5.,3.8));
#20115=CARTESIAN_POINT('',(13.4,3.4,12.7));
#20116=CARTESIAN_POINT('Origin',(13.4,5.,3.8));
#20117=CARTESIAN_POINT('',(8.6,5.,12.7));
#20118=CARTESIAN_POINT('',(8.6,5.,3.8));
#20119=CARTESIAN_POINT('',(13.4,5.,12.7));
#20120=CARTESIAN_POINT('',(7.4,5.,3.8));
#20121=CARTESIAN_POINT('Origin',(8.6,5.,3.8));
#20122=CARTESIAN_POINT('',(8.6,5.,12.7));
#20123=CARTESIAN_POINT('Origin',(11.,4.2,12.7));
#20124=CARTESIAN_POINT('Origin',(11.,4.2,3.8));
#34757=UNCERTAINTY_MEASURE_WITH_UNIT(LENGTH_MEASURE(0.001),#34852,
'DISTANCE_ACCURACY_VALUE',
'Maximum model space distance between geometric entities at asserted c
onnectivities');
#34797=UNCERTAINTY_MEASURE_WITH_UNIT(LENGTH_MEASURE(0.001),#34852,
'DISTANCE_ACCURACY_VALUE',
'Maximum model space distance between geometric entities at asserted c
onnectivities');
#34811=(
GEOMETRIC_REPRESENTATION_CONTEXT(3)
GLOBAL_UNCERTAINTY_ASSIGNED_CONTEXT((#34757))
GLOBAL_UNIT_ASSIGNED_CONTEXT((#34852,#34854,#34855))
REPRESENTATION_CONTEXT('','3D')
);
#34851=(
GEOMETRIC_REPRESENTATION_CONTEXT(3)
GLOBAL_UNCERTAINTY_ASSIGNED_CONTEXT((#34797))
GLOBAL_UNIT_ASSIGNED_CONTEXT((#34852,#34854,#34855))
REPRESENTATION_CONTEXT('','3D')
);
#34852=(
LENGTH_UNIT()
NAMED_UNIT(*)
SI_UNIT(.CENTI.,.METRE.)
);
#34854=(
NAMED_UNIT(*)
PLANE_ANGLE_UNIT()
SI_UNIT($,.RADIAN.)
);
#34855=(
NAMED_UNIT(*)
SI_UNIT($,.STERADIAN.)
SOLID_ANGLE_UNIT()
);
#34869=SHAPE_DEFINITION_REPRESENTATION(#34922,#35086);
#34922=PRODUCT_DEFINITION_SHAPE('',$,#35140);
#35086=SHAPE_REPRESENTATION('',(#14545),#34811);
#35126=PRODUCT_DEFINITION_CONTEXT('part definition',#35287,'design');
#35140=PRODUCT_DEFINITION('Pinion bearing pedestal (1)',
'Pinion bearing pedestal (1)',#35193,#35126);
#35193=PRODUCT_DEFINITION_FORMATION('',$,#35302);
#35287=APPLICATION_CONTEXT(
'Core Data for Automotive Mechanical Design Process');
#35288=PRODUCT_CONTEXT('part definition',#35287,'mechanical');
#35302=PRODUCT('Pinion bearing pedestal (1)',
'Pinion bearing pedestal (1)','Pinion bearing pedestal (1)',(#35288));
#35405=COLOUR_RGB('Grey',0.48,0.52,0.57);
#35406=FILL_AREA_STYLE_COLOUR('',#35405);
#35407=FILL_AREA_STYLE('',(#35406));
#35408=SURFACE_STYLE_FILL_AREA(#35407);
#35409=SURFACE_SIDE_STYLE('',(#35408));
#35410=SURFACE_STYLE_USAGE(.BOTH.,#35409);
#35411=PRESENTATION_STYLE_ASSIGNMENT((#35410));
ENDSEC;
END-ISO-10303-21;
